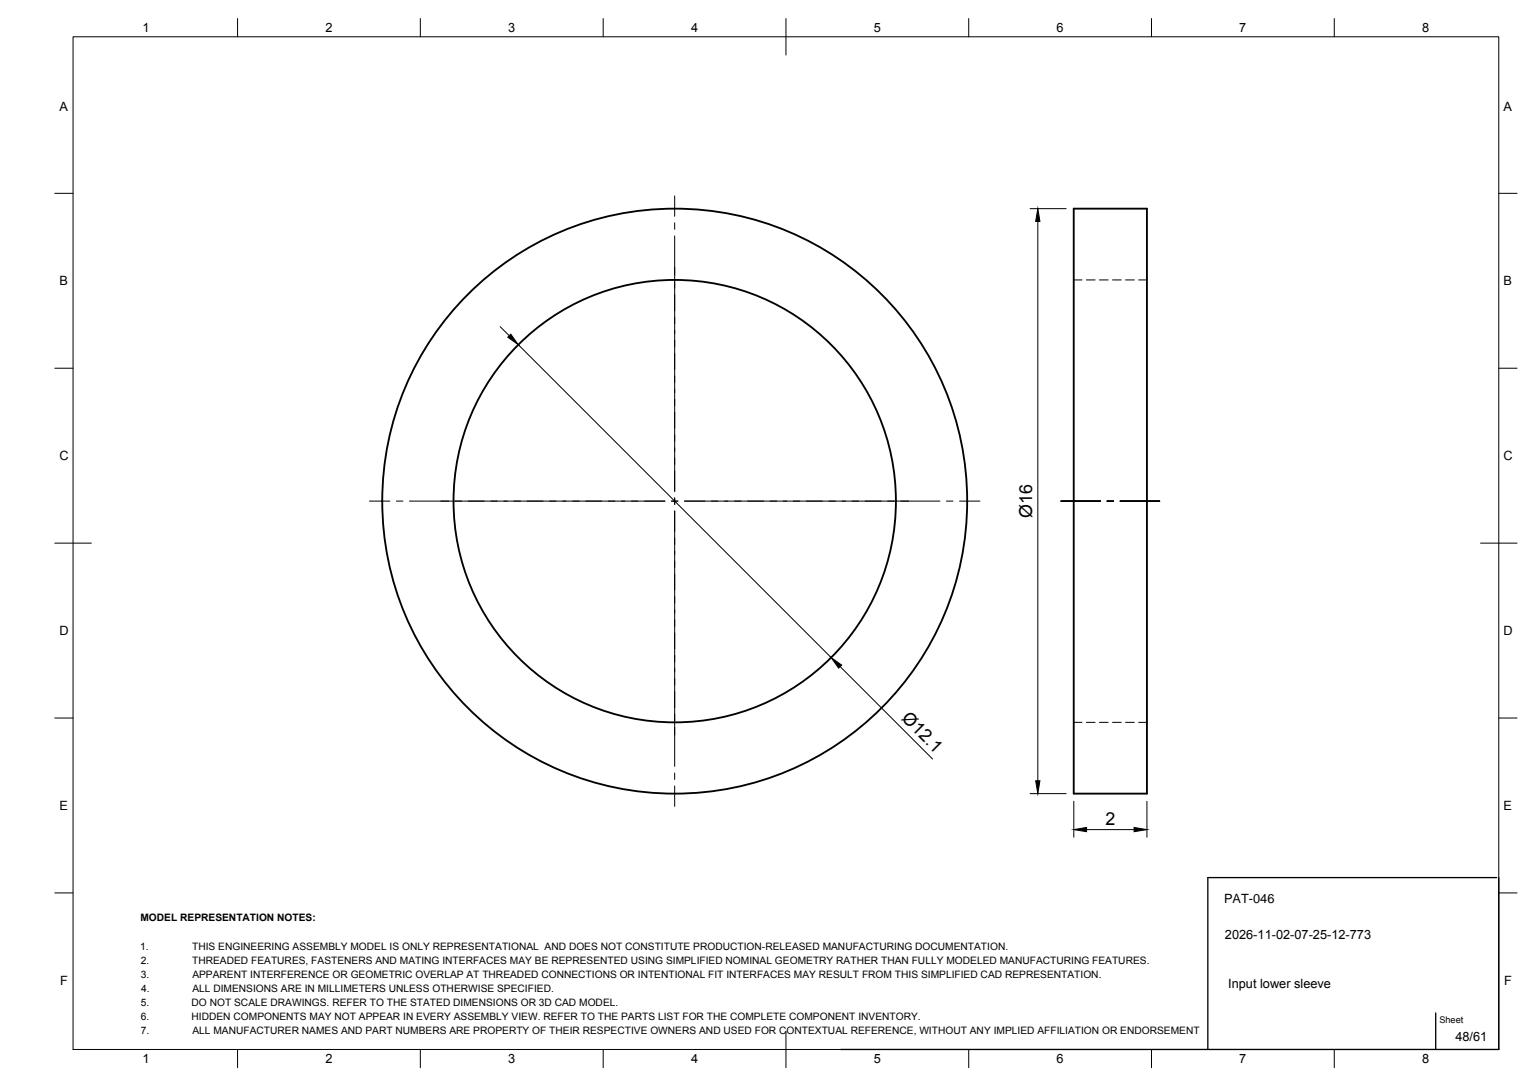
ISO-10303-21;
HEADER;
/* Generated by software containing ST-Developer
 * from STEP Tools, Inc. (www.steptools.com) 
 */

FILE_DESCRIPTION(
/* description */ ('Gear mesh backlash fixture'),
/* implementation_level */ '2;1');

FILE_NAME(
/* name */ 'Input lower sleeve.step',
/* time_stamp */ '2026-10-28T03:26:00-07:00',
/* author */ (''),
/* organization */ (''),
/* preprocessor_version */ 'ST-DEVELOPER v20.2',
/* originating_system */ 'Autodesk Translation Framework v15.17.0.0',
/* authorisation */ '');

FILE_SCHEMA (('AUTOMOTIVE_DESIGN { 1 0 10303 214 3 1 1 }'));
ENDSEC;

DATA;
#10=MECHANICAL_DESIGN_GEOMETRIC_PRESENTATION_REPRESENTATION('',(#1067),#57900);
#952=SHAPE_REPRESENTATION_RELATIONSHIP('SRR','None',#58152,#1002);
#1002=ADVANCED_BREP_SHAPE_REPRESENTATION('',(#1130),#57885);
#1067=STYLED_ITEM('',(#58479),#1130);
#1130=MANIFOLD_SOLID_BREP('Body1',#13629);
#1299=FACE_BOUND('',#3041,.T.);
#1300=FACE_BOUND('',#3043,.T.);
#1563=PLANE('',#15092);
#1564=PLANE('',#15093);
#2117=FACE_OUTER_BOUND('',#3038,.T.);
#2118=FACE_OUTER_BOUND('',#3039,.T.);
#2119=FACE_OUTER_BOUND('',#3040,.T.);
#2120=FACE_OUTER_BOUND('',#3042,.T.);
#3038=EDGE_LOOP('',(#10759,#10760,#10761,#10762));
#3039=EDGE_LOOP('',(#10763,#10764,#10765,#10766));
#3040=EDGE_LOOP('',(#10767));
#3041=EDGE_LOOP('',(#10768));
#3042=EDGE_LOOP('',(#10769));
#3043=EDGE_LOOP('',(#10770));
#3897=LINE('',#22089,#4786);
#3898=LINE('',#22095,#4787);
#4786=VECTOR('',#17850,0.605);
#4787=VECTOR('',#17857,0.8);
#5600=CIRCLE('',#15087,0.605);
#5601=CIRCLE('',#15088,0.605);
#5602=CIRCLE('',#15090,0.8);
#5603=CIRCLE('',#15091,0.8);
#6418=VERTEX_POINT('',#22086);
#6419=VERTEX_POINT('',#22088);
#6420=VERTEX_POINT('',#22092);
#6421=VERTEX_POINT('',#22094);
#7966=EDGE_CURVE('',#6418,#6418,#5600,.T.);
#7967=EDGE_CURVE('',#6418,#6419,#3897,.T.);
#7968=EDGE_CURVE('',#6419,#6419,#5601,.T.);
#7969=EDGE_CURVE('',#6420,#6420,#5602,.T.);
#7970=EDGE_CURVE('',#6420,#6421,#3898,.T.);
#7971=EDGE_CURVE('',#6421,#6421,#5603,.T.);
#10759=ORIENTED_EDGE('',*,*,#7966,.F.);
#10760=ORIENTED_EDGE('',*,*,#7967,.T.);
#10761=ORIENTED_EDGE('',*,*,#7968,.T.);
#10762=ORIENTED_EDGE('',*,*,#7967,.F.);
#10763=ORIENTED_EDGE('',*,*,#7969,.F.);
#10764=ORIENTED_EDGE('',*,*,#7970,.T.);
#10765=ORIENTED_EDGE('',*,*,#7971,.T.);
#10766=ORIENTED_EDGE('',*,*,#7970,.F.);
#10767=ORIENTED_EDGE('',*,*,#7969,.T.);
#10768=ORIENTED_EDGE('',*,*,#7966,.T.);
#10769=ORIENTED_EDGE('',*,*,#7971,.F.);
#10770=ORIENTED_EDGE('',*,*,#7968,.F.);
#12724=CYLINDRICAL_SURFACE('',#15086,0.605);
#12725=CYLINDRICAL_SURFACE('',#15089,0.8);
#13234=ADVANCED_FACE('',(#2117),#12724,.F.);
#13235=ADVANCED_FACE('',(#2118),#12725,.T.);
#13236=ADVANCED_FACE('',(#2119,#1299),#1563,.T.);
#13237=ADVANCED_FACE('',(#2120,#1300),#1564,.F.);
#13629=CLOSED_SHELL('',(#13234,#13235,#13236,#13237));
#15085=AXIS2_PLACEMENT_3D('',#22084,#17844,#17845);
#15086=AXIS2_PLACEMENT_3D('',#22085,#17846,#17847);
#15087=AXIS2_PLACEMENT_3D('',#22087,#17848,#17849);
#15088=AXIS2_PLACEMENT_3D('',#22090,#17851,#17852);
#15089=AXIS2_PLACEMENT_3D('',#22091,#17853,#17854);
#15090=AXIS2_PLACEMENT_3D('',#22093,#17855,#17856);
#15091=AXIS2_PLACEMENT_3D('',#22096,#17858,#17859);
#15092=AXIS2_PLACEMENT_3D('',#22097,#17860,#17861);
#15093=AXIS2_PLACEMENT_3D('',#22098,#17862,#17863);
#17844=DIRECTION('axis',(0.,0.,1.));
#17845=DIRECTION('refdir',(1.,0.,0.));
#17846=DIRECTION('center_axis',(0.,0.,1.));
#17847=DIRECTION('ref_axis',(1.,0.,0.));
#17848=DIRECTION('center_axis',(0.,0.,-1.));
#17849=DIRECTION('ref_axis',(1.,0.,0.));
#17850=DIRECTION('',(0.,0.,-1.));
#17851=DIRECTION('center_axis',(0.,0.,-1.));
#17852=DIRECTION('ref_axis',(1.,0.,0.));
#17853=DIRECTION('center_axis',(0.,0.,1.));
#17854=DIRECTION('ref_axis',(1.,0.,0.));
#17855=DIRECTION('center_axis',(0.,0.,1.));
#17856=DIRECTION('ref_axis',(1.,0.,0.));
#17857=DIRECTION('',(0.,0.,-1.));
#17858=DIRECTION('center_axis',(0.,0.,1.));
#17859=DIRECTION('ref_axis',(1.,0.,0.));
#17860=DIRECTION('center_axis',(0.,0.,1.));
#17861=DIRECTION('ref_axis',(1.,0.,0.));
#17862=DIRECTION('center_axis',(0.,0.,1.));
#17863=DIRECTION('ref_axis',(1.,0.,0.));
#22084=CARTESIAN_POINT('',(0.,0.,0.));
#22085=CARTESIAN_POINT('Origin',(0.,0.,5.8));
#22086=CARTESIAN_POINT('',(-0.605,-7.40911313484149E-17,6.));
#22087=CARTESIAN_POINT('Origin',(0.,0.,6.));
#22088=CARTESIAN_POINT('',(-0.605,-7.40911313484149E-17,5.8));
#22089=CARTESIAN_POINT('',(-0.605,-7.40911313484149E-17,5.8));
#22090=CARTESIAN_POINT('Origin',(0.,0.,5.8));
#22091=CARTESIAN_POINT('Origin',(0.,0.,5.8));
#22092=CARTESIAN_POINT('',(-0.8,-9.79717439317883E-17,6.));
#22093=CARTESIAN_POINT('Origin',(0.,0.,6.));
#22094=CARTESIAN_POINT('',(-0.8,-9.79717439317883E-17,5.8));
#22095=CARTESIAN_POINT('',(-0.8,-9.79717439317883E-17,5.8));
#22096=CARTESIAN_POINT('Origin',(0.,0.,5.8));
#22097=CARTESIAN_POINT('Origin',(0.,0.,6.));
#22098=CARTESIAN_POINT('Origin',(0.,0.,5.8));
#57826=UNCERTAINTY_MEASURE_WITH_UNIT(LENGTH_MEASURE(0.001),#57901,
'DISTANCE_ACCURACY_VALUE',
'Maximum model space distance between geometric entities at asserted c
onnectivities');
#57841=UNCERTAINTY_MEASURE_WITH_UNIT(LENGTH_MEASURE(0.001),#57901,
'DISTANCE_ACCURACY_VALUE',
'Maximum model space distance between geometric entities at asserted c
onnectivities');
#57885=(
GEOMETRIC_REPRESENTATION_CONTEXT(3)
GLOBAL_UNCERTAINTY_ASSIGNED_CONTEXT((#57826))
GLOBAL_UNIT_ASSIGNED_CONTEXT((#57901,#57903,#57904))
REPRESENTATION_CONTEXT('','3D')
);
#57900=(
GEOMETRIC_REPRESENTATION_CONTEXT(3)
GLOBAL_UNCERTAINTY_ASSIGNED_CONTEXT((#57841))
GLOBAL_UNIT_ASSIGNED_CONTEXT((#57901,#57903,#57904))
REPRESENTATION_CONTEXT('','3D')
);
#57901=(
LENGTH_UNIT()
NAMED_UNIT(*)
SI_UNIT(.CENTI.,.METRE.)
);
#57903=(
NAMED_UNIT(*)
PLANE_ANGLE_UNIT()
SI_UNIT($,.RADIAN.)
);
#57904=(
NAMED_UNIT(*)
SI_UNIT($,.STERADIAN.)
SOLID_ANGLE_UNIT()
);
#57948=SHAPE_DEFINITION_REPRESENTATION(#58019,#58152);
#58019=PRODUCT_DEFINITION_SHAPE('',$,#58211);
#58152=SHAPE_REPRESENTATION('',(#15085),#57885);
#58167=PRODUCT_DEFINITION_CONTEXT('part definition',#58343,'design');
#58211=PRODUCT_DEFINITION('Input lower sleeve','Input lower sleeve',#58269,
#58167);
#58269=PRODUCT_DEFINITION_FORMATION('',$,#58388);
#58343=APPLICATION_CONTEXT(
'Core Data for Automotive Mechanical Design Process');
#58344=PRODUCT_CONTEXT('part definition',#58343,'mechanical');
#58388=PRODUCT('Input lower sleeve','Input lower sleeve',
'Input lower sleeve',(#58344));
#58473=COLOUR_RGB('Off White',0.89,0.88,0.83);
#58474=FILL_AREA_STYLE_COLOUR('',#58473);
#58475=FILL_AREA_STYLE('',(#58474));
#58476=SURFACE_STYLE_FILL_AREA(#58475);
#58477=SURFACE_SIDE_STYLE('',(#58476));
#58478=SURFACE_STYLE_USAGE(.BOTH.,#58477);
#58479=PRESENTATION_STYLE_ASSIGNMENT((#58478));
ENDSEC;
END-ISO-10303-21;
